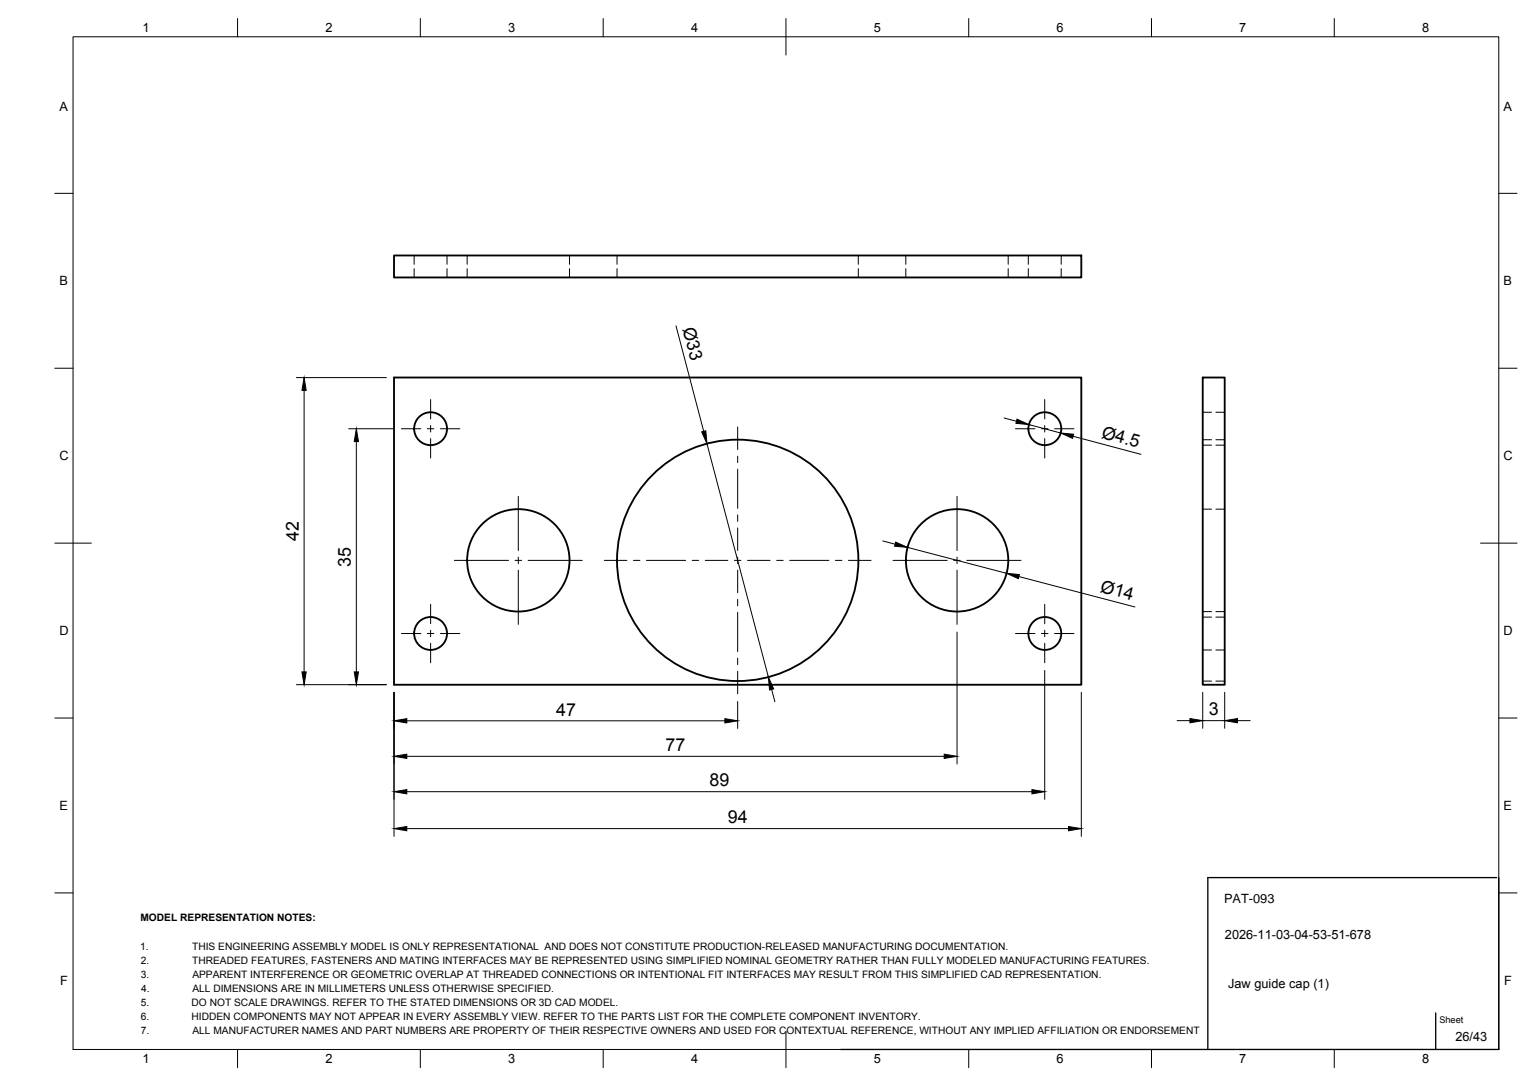
ISO-10303-21;
HEADER;
/* Generated by software containing ST-Developer
 * from STEP Tools, Inc. (www.steptools.com) 
 */

FILE_DESCRIPTION(
/* description */ ('Self-centering screw clamp'),
/* implementation_level */ '2;1');

FILE_NAME(
/* name */ 'Jaw guide cap (1).step',
/* time_stamp */ '2026-10-28T03:25:31-07:00',
/* author */ (''),
/* organization */ (''),
/* preprocessor_version */ 'ST-DEVELOPER v20.2',
/* originating_system */ 'Autodesk Translation Framework v15.17.0.0',
/* authorisation */ '');

FILE_SCHEMA (('AUTOMOTIVE_DESIGN { 1 0 10303 214 3 1 1 }'));
ENDSEC;

DATA;
#10=MECHANICAL_DESIGN_GEOMETRIC_PRESENTATION_REPRESENTATION('',(#652),#16799);
#563=SHAPE_REPRESENTATION_RELATIONSHIP('SRR','None',#17038,#604);
#604=ADVANCED_BREP_SHAPE_REPRESENTATION('',(#700),#16776);
#652=STYLED_ITEM('',(#17312),#700);
#700=MANIFOLD_SOLID_BREP('Body1',#9103);
#885=FACE_BOUND('',#2220,.T.);
#886=FACE_BOUND('',#2221,.T.);
#887=FACE_BOUND('',#2222,.T.);
#888=FACE_BOUND('',#2223,.T.);
#889=FACE_BOUND('',#2224,.T.);
#890=FACE_BOUND('',#2225,.T.);
#891=FACE_BOUND('',#2226,.T.);
#892=FACE_BOUND('',#2229,.T.);
#893=FACE_BOUND('',#2230,.T.);
#894=FACE_BOUND('',#2231,.T.);
#895=FACE_BOUND('',#2232,.T.);
#896=FACE_BOUND('',#2233,.T.);
#897=FACE_BOUND('',#2234,.T.);
#898=FACE_BOUND('',#2235,.T.);
#1140=PLANE('',#10185);
#1141=PLANE('',#10186);
#1142=PLANE('',#10187);
#1143=PLANE('',#10188);
#1144=PLANE('',#10189);
#1145=PLANE('',#10190);
#1540=FACE_OUTER_BOUND('',#2211,.T.);
#1541=FACE_OUTER_BOUND('',#2212,.T.);
#1542=FACE_OUTER_BOUND('',#2213,.T.);
#1543=FACE_OUTER_BOUND('',#2214,.T.);
#1544=FACE_OUTER_BOUND('',#2215,.T.);
#1545=FACE_OUTER_BOUND('',#2216,.T.);
#1546=FACE_OUTER_BOUND('',#2217,.T.);
#1547=FACE_OUTER_BOUND('',#2218,.T.);
#1548=FACE_OUTER_BOUND('',#2219,.T.);
#1549=FACE_OUTER_BOUND('',#2227,.T.);
#1550=FACE_OUTER_BOUND('',#2228,.T.);
#1551=FACE_OUTER_BOUND('',#2236,.T.);
#1552=FACE_OUTER_BOUND('',#2237,.T.);
#2211=EDGE_LOOP('',(#7359,#7360,#7361,#7362));
#2212=EDGE_LOOP('',(#7363,#7364,#7365,#7366));
#2213=EDGE_LOOP('',(#7367,#7368,#7369,#7370));
#2214=EDGE_LOOP('',(#7371,#7372,#7373,#7374));
#2215=EDGE_LOOP('',(#7375,#7376,#7377,#7378));
#2216=EDGE_LOOP('',(#7379,#7380,#7381,#7382));
#2217=EDGE_LOOP('',(#7383,#7384,#7385,#7386));
#2218=EDGE_LOOP('',(#7387,#7388,#7389,#7390));
#2219=EDGE_LOOP('',(#7391,#7392,#7393,#7394));
#2220=EDGE_LOOP('',(#7395));
#2221=EDGE_LOOP('',(#7396));
#2222=EDGE_LOOP('',(#7397));
#2223=EDGE_LOOP('',(#7398));
#2224=EDGE_LOOP('',(#7399));
#2225=EDGE_LOOP('',(#7400));
#2226=EDGE_LOOP('',(#7401));
#2227=EDGE_LOOP('',(#7402,#7403,#7404,#7405));
#2228=EDGE_LOOP('',(#7406,#7407,#7408,#7409));
#2229=EDGE_LOOP('',(#7410));
#2230=EDGE_LOOP('',(#7411));
#2231=EDGE_LOOP('',(#7412));
#2232=EDGE_LOOP('',(#7413));
#2233=EDGE_LOOP('',(#7414));
#2234=EDGE_LOOP('',(#7415));
#2235=EDGE_LOOP('',(#7416));
#2236=EDGE_LOOP('',(#7417,#7418,#7419,#7420));
#2237=EDGE_LOOP('',(#7421,#7422,#7423,#7424));
#2886=LINE('',#15393,#3459);
#2887=LINE('',#15399,#3460);
#2888=LINE('',#15405,#3461);
#2889=LINE('',#15411,#3462);
#2890=LINE('',#15417,#3463);
#2891=LINE('',#15423,#3464);
#2892=LINE('',#15429,#3465);
#2893=LINE('',#15434,#3466);
#2894=LINE('',#15436,#3467);
#2895=LINE('',#15438,#3468);
#2896=LINE('',#15439,#3469);
#2897=LINE('',#15442,#3470);
#2898=LINE('',#15444,#3471);
#2899=LINE('',#15445,#3472);
#2900=LINE('',#15448,#3473);
#2901=LINE('',#15450,#3474);
#2902=LINE('',#15451,#3475);
#2903=LINE('',#15453,#3476);
#2904=LINE('',#15454,#3477);
#3459=VECTOR('',#12239,0.225);
#3460=VECTOR('',#12246,0.225);
#3461=VECTOR('',#12253,0.225);
#3462=VECTOR('',#12260,0.225);
#3463=VECTOR('',#12267,1.65);
#3464=VECTOR('',#12274,0.7);
#3465=VECTOR('',#12281,0.7);
#3466=VECTOR('',#12286,1.);
#3467=VECTOR('',#12287,1.);
#3468=VECTOR('',#12288,1.);
#3469=VECTOR('',#12289,1.);
#3470=VECTOR('',#12292,1.);
#3471=VECTOR('',#12293,1.);
#3472=VECTOR('',#12294,1.);
#3473=VECTOR('',#12297,1.);
#3474=VECTOR('',#12298,1.);
#3475=VECTOR('',#12299,1.);
#3476=VECTOR('',#12302,1.);
#3477=VECTOR('',#12303,1.);
#4012=CIRCLE('',#10165,0.225);
#4013=CIRCLE('',#10166,0.225);
#4014=CIRCLE('',#10168,0.225);
#4015=CIRCLE('',#10169,0.225);
#4016=CIRCLE('',#10171,0.225);
#4017=CIRCLE('',#10172,0.225);
#4018=CIRCLE('',#10174,0.225);
#4019=CIRCLE('',#10175,0.225);
#4020=CIRCLE('',#10177,1.65);
#4021=CIRCLE('',#10178,1.65);
#4022=CIRCLE('',#10180,0.7);
#4023=CIRCLE('',#10181,0.7);
#4024=CIRCLE('',#10183,0.7);
#4025=CIRCLE('',#10184,0.7);
#4647=VERTEX_POINT('',#15390);
#4648=VERTEX_POINT('',#15392);
#4649=VERTEX_POINT('',#15396);
#4650=VERTEX_POINT('',#15398);
#4651=VERTEX_POINT('',#15402);
#4652=VERTEX_POINT('',#15404);
#4653=VERTEX_POINT('',#15408);
#4654=VERTEX_POINT('',#15410);
#4655=VERTEX_POINT('',#15414);
#4656=VERTEX_POINT('',#15416);
#4657=VERTEX_POINT('',#15420);
#4658=VERTEX_POINT('',#15422);
#4659=VERTEX_POINT('',#15426);
#4660=VERTEX_POINT('',#15428);
#4661=VERTEX_POINT('',#15432);
#4662=VERTEX_POINT('',#15433);
#4663=VERTEX_POINT('',#15435);
#4664=VERTEX_POINT('',#15437);
#4665=VERTEX_POINT('',#15441);
#4666=VERTEX_POINT('',#15443);
#4667=VERTEX_POINT('',#15447);
#4668=VERTEX_POINT('',#15449);
#5604=EDGE_CURVE('',#4647,#4647,#4012,.T.);
#5605=EDGE_CURVE('',#4647,#4648,#2886,.T.);
#5606=EDGE_CURVE('',#4648,#4648,#4013,.T.);
#5607=EDGE_CURVE('',#4649,#4649,#4014,.T.);
#5608=EDGE_CURVE('',#4649,#4650,#2887,.T.);
#5609=EDGE_CURVE('',#4650,#4650,#4015,.T.);
#5610=EDGE_CURVE('',#4651,#4651,#4016,.T.);
#5611=EDGE_CURVE('',#4651,#4652,#2888,.T.);
#5612=EDGE_CURVE('',#4652,#4652,#4017,.T.);
#5613=EDGE_CURVE('',#4653,#4653,#4018,.T.);
#5614=EDGE_CURVE('',#4653,#4654,#2889,.T.);
#5615=EDGE_CURVE('',#4654,#4654,#4019,.T.);
#5616=EDGE_CURVE('',#4655,#4655,#4020,.T.);
#5617=EDGE_CURVE('',#4655,#4656,#2890,.T.);
#5618=EDGE_CURVE('',#4656,#4656,#4021,.T.);
#5619=EDGE_CURVE('',#4657,#4657,#4022,.T.);
#5620=EDGE_CURVE('',#4657,#4658,#2891,.T.);
#5621=EDGE_CURVE('',#4658,#4658,#4023,.T.);
#5622=EDGE_CURVE('',#4659,#4659,#4024,.T.);
#5623=EDGE_CURVE('',#4659,#4660,#2892,.T.);
#5624=EDGE_CURVE('',#4660,#4660,#4025,.T.);
#5625=EDGE_CURVE('',#4661,#4662,#2893,.T.);
#5626=EDGE_CURVE('',#4662,#4663,#2894,.T.);
#5627=EDGE_CURVE('',#4664,#4663,#2895,.T.);
#5628=EDGE_CURVE('',#4661,#4664,#2896,.T.);
#5629=EDGE_CURVE('',#4665,#4661,#2897,.T.);
#5630=EDGE_CURVE('',#4666,#4664,#2898,.T.);
#5631=EDGE_CURVE('',#4665,#4666,#2899,.T.);
#5632=EDGE_CURVE('',#4667,#4665,#2900,.T.);
#5633=EDGE_CURVE('',#4668,#4666,#2901,.T.);
#5634=EDGE_CURVE('',#4667,#4668,#2902,.T.);
#5635=EDGE_CURVE('',#4662,#4667,#2903,.T.);
#5636=EDGE_CURVE('',#4663,#4668,#2904,.T.);
#7359=ORIENTED_EDGE('',*,*,#5604,.F.);
#7360=ORIENTED_EDGE('',*,*,#5605,.T.);
#7361=ORIENTED_EDGE('',*,*,#5606,.F.);
#7362=ORIENTED_EDGE('',*,*,#5605,.F.);
#7363=ORIENTED_EDGE('',*,*,#5607,.F.);
#7364=ORIENTED_EDGE('',*,*,#5608,.T.);
#7365=ORIENTED_EDGE('',*,*,#5609,.F.);
#7366=ORIENTED_EDGE('',*,*,#5608,.F.);
#7367=ORIENTED_EDGE('',*,*,#5610,.F.);
#7368=ORIENTED_EDGE('',*,*,#5611,.T.);
#7369=ORIENTED_EDGE('',*,*,#5612,.F.);
#7370=ORIENTED_EDGE('',*,*,#5611,.F.);
#7371=ORIENTED_EDGE('',*,*,#5613,.F.);
#7372=ORIENTED_EDGE('',*,*,#5614,.T.);
#7373=ORIENTED_EDGE('',*,*,#5615,.F.);
#7374=ORIENTED_EDGE('',*,*,#5614,.F.);
#7375=ORIENTED_EDGE('',*,*,#5616,.F.);
#7376=ORIENTED_EDGE('',*,*,#5617,.T.);
#7377=ORIENTED_EDGE('',*,*,#5618,.F.);
#7378=ORIENTED_EDGE('',*,*,#5617,.F.);
#7379=ORIENTED_EDGE('',*,*,#5619,.F.);
#7380=ORIENTED_EDGE('',*,*,#5620,.T.);
#7381=ORIENTED_EDGE('',*,*,#5621,.F.);
#7382=ORIENTED_EDGE('',*,*,#5620,.F.);
#7383=ORIENTED_EDGE('',*,*,#5622,.F.);
#7384=ORIENTED_EDGE('',*,*,#5623,.T.);
#7385=ORIENTED_EDGE('',*,*,#5624,.F.);
#7386=ORIENTED_EDGE('',*,*,#5623,.F.);
#7387=ORIENTED_EDGE('',*,*,#5625,.T.);
#7388=ORIENTED_EDGE('',*,*,#5626,.T.);
#7389=ORIENTED_EDGE('',*,*,#5627,.F.);
#7390=ORIENTED_EDGE('',*,*,#5628,.F.);
#7391=ORIENTED_EDGE('',*,*,#5629,.T.);
#7392=ORIENTED_EDGE('',*,*,#5628,.T.);
#7393=ORIENTED_EDGE('',*,*,#5630,.F.);
#7394=ORIENTED_EDGE('',*,*,#5631,.F.);
#7395=ORIENTED_EDGE('',*,*,#5624,.T.);
#7396=ORIENTED_EDGE('',*,*,#5621,.T.);
#7397=ORIENTED_EDGE('',*,*,#5618,.T.);
#7398=ORIENTED_EDGE('',*,*,#5615,.T.);
#7399=ORIENTED_EDGE('',*,*,#5612,.T.);
#7400=ORIENTED_EDGE('',*,*,#5609,.T.);
#7401=ORIENTED_EDGE('',*,*,#5606,.T.);
#7402=ORIENTED_EDGE('',*,*,#5632,.T.);
#7403=ORIENTED_EDGE('',*,*,#5631,.T.);
#7404=ORIENTED_EDGE('',*,*,#5633,.F.);
#7405=ORIENTED_EDGE('',*,*,#5634,.F.);
#7406=ORIENTED_EDGE('',*,*,#5635,.T.);
#7407=ORIENTED_EDGE('',*,*,#5634,.T.);
#7408=ORIENTED_EDGE('',*,*,#5636,.F.);
#7409=ORIENTED_EDGE('',*,*,#5626,.F.);
#7410=ORIENTED_EDGE('',*,*,#5622,.T.);
#7411=ORIENTED_EDGE('',*,*,#5619,.T.);
#7412=ORIENTED_EDGE('',*,*,#5616,.T.);
#7413=ORIENTED_EDGE('',*,*,#5613,.T.);
#7414=ORIENTED_EDGE('',*,*,#5610,.T.);
#7415=ORIENTED_EDGE('',*,*,#5607,.T.);
#7416=ORIENTED_EDGE('',*,*,#5604,.T.);
#7417=ORIENTED_EDGE('',*,*,#5636,.T.);
#7418=ORIENTED_EDGE('',*,*,#5633,.T.);
#7419=ORIENTED_EDGE('',*,*,#5630,.T.);
#7420=ORIENTED_EDGE('',*,*,#5627,.T.);
#7421=ORIENTED_EDGE('',*,*,#5635,.F.);
#7422=ORIENTED_EDGE('',*,*,#5625,.F.);
#7423=ORIENTED_EDGE('',*,*,#5629,.F.);
#7424=ORIENTED_EDGE('',*,*,#5632,.F.);
#8476=CYLINDRICAL_SURFACE('',#10164,0.225);
#8477=CYLINDRICAL_SURFACE('',#10167,0.225);
#8478=CYLINDRICAL_SURFACE('',#10170,0.225);
#8479=CYLINDRICAL_SURFACE('',#10173,0.225);
#8480=CYLINDRICAL_SURFACE('',#10176,1.65);
#8481=CYLINDRICAL_SURFACE('',#10179,0.7);
#8482=CYLINDRICAL_SURFACE('',#10182,0.7);
#8838=ADVANCED_FACE('',(#1540),#8476,.F.);
#8839=ADVANCED_FACE('',(#1541),#8477,.F.);
#8840=ADVANCED_FACE('',(#1542),#8478,.F.);
#8841=ADVANCED_FACE('',(#1543),#8479,.F.);
#8842=ADVANCED_FACE('',(#1544),#8480,.F.);
#8843=ADVANCED_FACE('',(#1545),#8481,.F.);
#8844=ADVANCED_FACE('',(#1546),#8482,.F.);
#8845=ADVANCED_FACE('',(#1547),#1140,.T.);
#8846=ADVANCED_FACE('',(#1548,#885,#886,#887,#888,#889,#890,#891),#1141,
 .T.);
#8847=ADVANCED_FACE('',(#1549),#1142,.T.);
#8848=ADVANCED_FACE('',(#1550,#892,#893,#894,#895,#896,#897,#898),#1143,
 .T.);
#8849=ADVANCED_FACE('',(#1551),#1144,.T.);
#8850=ADVANCED_FACE('',(#1552),#1145,.F.);
#9103=CLOSED_SHELL('',(#8838,#8839,#8840,#8841,#8842,#8843,#8844,#8845,
#8846,#8847,#8848,#8849,#8850));
#10163=AXIS2_PLACEMENT_3D('',#15388,#12233,#12234);
#10164=AXIS2_PLACEMENT_3D('',#15389,#12235,#12236);
#10165=AXIS2_PLACEMENT_3D('',#15391,#12237,#12238);
#10166=AXIS2_PLACEMENT_3D('',#15394,#12240,#12241);
#10167=AXIS2_PLACEMENT_3D('',#15395,#12242,#12243);
#10168=AXIS2_PLACEMENT_3D('',#15397,#12244,#12245);
#10169=AXIS2_PLACEMENT_3D('',#15400,#12247,#12248);
#10170=AXIS2_PLACEMENT_3D('',#15401,#12249,#12250);
#10171=AXIS2_PLACEMENT_3D('',#15403,#12251,#12252);
#10172=AXIS2_PLACEMENT_3D('',#15406,#12254,#12255);
#10173=AXIS2_PLACEMENT_3D('',#15407,#12256,#12257);
#10174=AXIS2_PLACEMENT_3D('',#15409,#12258,#12259);
#10175=AXIS2_PLACEMENT_3D('',#15412,#12261,#12262);
#10176=AXIS2_PLACEMENT_3D('',#15413,#12263,#12264);
#10177=AXIS2_PLACEMENT_3D('',#15415,#12265,#12266);
#10178=AXIS2_PLACEMENT_3D('',#15418,#12268,#12269);
#10179=AXIS2_PLACEMENT_3D('',#15419,#12270,#12271);
#10180=AXIS2_PLACEMENT_3D('',#15421,#12272,#12273);
#10181=AXIS2_PLACEMENT_3D('',#15424,#12275,#12276);
#10182=AXIS2_PLACEMENT_3D('',#15425,#12277,#12278);
#10183=AXIS2_PLACEMENT_3D('',#15427,#12279,#12280);
#10184=AXIS2_PLACEMENT_3D('',#15430,#12282,#12283);
#10185=AXIS2_PLACEMENT_3D('',#15431,#12284,#12285);
#10186=AXIS2_PLACEMENT_3D('',#15440,#12290,#12291);
#10187=AXIS2_PLACEMENT_3D('',#15446,#12295,#12296);
#10188=AXIS2_PLACEMENT_3D('',#15452,#12300,#12301);
#10189=AXIS2_PLACEMENT_3D('',#15455,#12304,#12305);
#10190=AXIS2_PLACEMENT_3D('',#15456,#12306,#12307);
#12233=DIRECTION('axis',(0.,0.,1.));
#12234=DIRECTION('refdir',(1.,0.,0.));
#12235=DIRECTION('center_axis',(1.,0.,0.));
#12236=DIRECTION('ref_axis',(0.,0.,-1.));
#12237=DIRECTION('center_axis',(1.,0.,0.));
#12238=DIRECTION('ref_axis',(0.,0.,-1.));
#12239=DIRECTION('',(1.,0.,0.));
#12240=DIRECTION('center_axis',(-1.,0.,0.));
#12241=DIRECTION('ref_axis',(0.,0.,-1.));
#12242=DIRECTION('center_axis',(1.,0.,0.));
#12243=DIRECTION('ref_axis',(0.,0.,-1.));
#12244=DIRECTION('center_axis',(1.,0.,0.));
#12245=DIRECTION('ref_axis',(0.,0.,-1.));
#12246=DIRECTION('',(1.,0.,0.));
#12247=DIRECTION('center_axis',(-1.,0.,0.));
#12248=DIRECTION('ref_axis',(0.,0.,-1.));
#12249=DIRECTION('center_axis',(1.,0.,0.));
#12250=DIRECTION('ref_axis',(0.,0.,-1.));
#12251=DIRECTION('center_axis',(1.,0.,0.));
#12252=DIRECTION('ref_axis',(0.,0.,-1.));
#12253=DIRECTION('',(1.,0.,0.));
#12254=DIRECTION('center_axis',(-1.,0.,0.));
#12255=DIRECTION('ref_axis',(0.,0.,-1.));
#12256=DIRECTION('center_axis',(1.,0.,0.));
#12257=DIRECTION('ref_axis',(0.,0.,-1.));
#12258=DIRECTION('center_axis',(1.,0.,0.));
#12259=DIRECTION('ref_axis',(0.,0.,-1.));
#12260=DIRECTION('',(1.,0.,0.));
#12261=DIRECTION('center_axis',(-1.,0.,0.));
#12262=DIRECTION('ref_axis',(0.,0.,-1.));
#12263=DIRECTION('center_axis',(1.,0.,0.));
#12264=DIRECTION('ref_axis',(0.,0.,-1.));
#12265=DIRECTION('center_axis',(1.,0.,0.));
#12266=DIRECTION('ref_axis',(0.,0.,-1.));
#12267=DIRECTION('',(1.,0.,0.));
#12268=DIRECTION('center_axis',(-1.,0.,0.));
#12269=DIRECTION('ref_axis',(0.,0.,-1.));
#12270=DIRECTION('center_axis',(1.,0.,0.));
#12271=DIRECTION('ref_axis',(0.,0.,-1.));
#12272=DIRECTION('center_axis',(1.,0.,0.));
#12273=DIRECTION('ref_axis',(0.,0.,-1.));
#12274=DIRECTION('',(1.,0.,0.));
#12275=DIRECTION('center_axis',(-1.,0.,0.));
#12276=DIRECTION('ref_axis',(0.,0.,-1.));
#12277=DIRECTION('center_axis',(1.,0.,0.));
#12278=DIRECTION('ref_axis',(0.,0.,-1.));
#12279=DIRECTION('center_axis',(1.,0.,0.));
#12280=DIRECTION('ref_axis',(0.,0.,-1.));
#12281=DIRECTION('',(1.,0.,0.));
#12282=DIRECTION('center_axis',(-1.,0.,0.));
#12283=DIRECTION('ref_axis',(0.,0.,-1.));
#12284=DIRECTION('center_axis',(0.,1.,0.));
#12285=DIRECTION('ref_axis',(-1.,0.,0.));
#12286=DIRECTION('',(-1.,0.,0.));
#12287=DIRECTION('',(0.,0.,1.));
#12288=DIRECTION('',(-1.,0.,0.));
#12289=DIRECTION('',(0.,0.,1.));
#12290=DIRECTION('center_axis',(1.,0.,0.));
#12291=DIRECTION('ref_axis',(0.,1.,0.));
#12292=DIRECTION('',(0.,1.,0.));
#12293=DIRECTION('',(0.,1.,0.));
#12294=DIRECTION('',(0.,0.,1.));
#12295=DIRECTION('center_axis',(0.,-1.,0.));
#12296=DIRECTION('ref_axis',(1.,0.,0.));
#12297=DIRECTION('',(1.,0.,0.));
#12298=DIRECTION('',(1.,0.,0.));
#12299=DIRECTION('',(0.,0.,1.));
#12300=DIRECTION('center_axis',(-1.,0.,0.));
#12301=DIRECTION('ref_axis',(0.,-1.,0.));
#12302=DIRECTION('',(0.,-1.,0.));
#12303=DIRECTION('',(0.,-1.,0.));
#12304=DIRECTION('center_axis',(0.,0.,1.));
#12305=DIRECTION('ref_axis',(1.,0.,0.));
#12306=DIRECTION('center_axis',(0.,0.,1.));
#12307=DIRECTION('ref_axis',(1.,0.,0.));
#15388=CARTESIAN_POINT('',(0.,0.,0.));
#15389=CARTESIAN_POINT('Origin',(-5.6,4.2,3.));
#15390=CARTESIAN_POINT('',(-5.5,4.2,3.225));
#15391=CARTESIAN_POINT('Origin',(-5.5,4.2,3.));
#15392=CARTESIAN_POINT('',(-5.2,4.2,3.225));
#15393=CARTESIAN_POINT('',(-5.6,4.2,3.225));
#15394=CARTESIAN_POINT('Origin',(-5.2,4.2,3.));
#15395=CARTESIAN_POINT('Origin',(-5.6,-4.2,5.8));
#15396=CARTESIAN_POINT('',(-5.5,-4.2,6.025));
#15397=CARTESIAN_POINT('Origin',(-5.5,-4.2,5.8));
#15398=CARTESIAN_POINT('',(-5.2,-4.2,6.025));
#15399=CARTESIAN_POINT('',(-5.6,-4.2,6.025));
#15400=CARTESIAN_POINT('Origin',(-5.2,-4.2,5.8));
#15401=CARTESIAN_POINT('Origin',(-5.6,-4.2,3.));
#15402=CARTESIAN_POINT('',(-5.5,-4.2,3.225));
#15403=CARTESIAN_POINT('Origin',(-5.5,-4.2,3.));
#15404=CARTESIAN_POINT('',(-5.2,-4.2,3.225));
#15405=CARTESIAN_POINT('',(-5.6,-4.2,3.225));
#15406=CARTESIAN_POINT('Origin',(-5.2,-4.2,3.));
#15407=CARTESIAN_POINT('Origin',(-5.6,4.2,5.8));
#15408=CARTESIAN_POINT('',(-5.5,4.2,6.025));
#15409=CARTESIAN_POINT('Origin',(-5.5,4.2,5.8));
#15410=CARTESIAN_POINT('',(-5.2,4.2,6.025));
#15411=CARTESIAN_POINT('',(-5.6,4.2,6.025));
#15412=CARTESIAN_POINT('Origin',(-5.2,4.2,5.8));
#15413=CARTESIAN_POINT('Origin',(-5.6,0.,4.));
#15414=CARTESIAN_POINT('',(-5.5,-2.02066721859313E-16,5.65));
#15415=CARTESIAN_POINT('Origin',(-5.5,0.,4.));
#15416=CARTESIAN_POINT('',(-5.2,2.02066721859313E-16,5.65));
#15417=CARTESIAN_POINT('',(-5.6,-2.02066721859313E-16,5.65));
#15418=CARTESIAN_POINT('Origin',(-5.2,0.,4.));
#15419=CARTESIAN_POINT('Origin',(-5.6,-3.,4.));
#15420=CARTESIAN_POINT('',(-5.5,-3.,4.7));
#15421=CARTESIAN_POINT('Origin',(-5.5,-3.,4.));
#15422=CARTESIAN_POINT('',(-5.2,-3.,4.7));
#15423=CARTESIAN_POINT('',(-5.6,-3.,4.7));
#15424=CARTESIAN_POINT('Origin',(-5.2,-3.,4.));
#15425=CARTESIAN_POINT('Origin',(-5.6,3.,4.));
#15426=CARTESIAN_POINT('',(-5.5,3.,4.7));
#15427=CARTESIAN_POINT('Origin',(-5.5,3.,4.));
#15428=CARTESIAN_POINT('',(-5.2,3.,4.7));
#15429=CARTESIAN_POINT('',(-5.6,3.,4.7));
#15430=CARTESIAN_POINT('Origin',(-5.2,3.,4.));
#15431=CARTESIAN_POINT('Origin',(-5.2,4.7,2.3));
#15432=CARTESIAN_POINT('',(-5.2,4.7,2.3));
#15433=CARTESIAN_POINT('',(-5.5,4.7,2.3));
#15434=CARTESIAN_POINT('',(-5.2,4.7,2.3));
#15435=CARTESIAN_POINT('',(-5.5,4.7,6.5));
#15436=CARTESIAN_POINT('',(-5.5,4.7,2.3));
#15437=CARTESIAN_POINT('',(-5.2,4.7,6.5));
#15438=CARTESIAN_POINT('',(-5.2,4.7,6.5));
#15439=CARTESIAN_POINT('',(-5.2,4.7,2.3));
#15440=CARTESIAN_POINT('Origin',(-5.2,-4.7,2.3));
#15441=CARTESIAN_POINT('',(-5.2,-4.7,2.3));
#15442=CARTESIAN_POINT('',(-5.2,-4.7,2.3));
#15443=CARTESIAN_POINT('',(-5.2,-4.7,6.5));
#15444=CARTESIAN_POINT('',(-5.2,-4.7,6.5));
#15445=CARTESIAN_POINT('',(-5.2,-4.7,2.3));
#15446=CARTESIAN_POINT('Origin',(-5.5,-4.7,2.3));
#15447=CARTESIAN_POINT('',(-5.5,-4.7,2.3));
#15448=CARTESIAN_POINT('',(-5.5,-4.7,2.3));
#15449=CARTESIAN_POINT('',(-5.5,-4.7,6.5));
#15450=CARTESIAN_POINT('',(-5.5,-4.7,6.5));
#15451=CARTESIAN_POINT('',(-5.5,-4.7,2.3));
#15452=CARTESIAN_POINT('Origin',(-5.5,4.7,2.3));
#15453=CARTESIAN_POINT('',(-5.5,4.7,2.3));
#15454=CARTESIAN_POINT('',(-5.5,4.7,6.5));
#15455=CARTESIAN_POINT('Origin',(-5.35,0.,6.5));
#15456=CARTESIAN_POINT('Origin',(-5.35,0.,2.3));
#16727=UNCERTAINTY_MEASURE_WITH_UNIT(LENGTH_MEASURE(0.001),#16800,
'DISTANCE_ACCURACY_VALUE',
'Maximum model space distance between geometric entities at asserted c
onnectivities');
#16750=UNCERTAINTY_MEASURE_WITH_UNIT(LENGTH_MEASURE(0.001),#16800,
'DISTANCE_ACCURACY_VALUE',
'Maximum model space distance between geometric entities at asserted c
onnectivities');
#16776=(
GEOMETRIC_REPRESENTATION_CONTEXT(3)
GLOBAL_UNCERTAINTY_ASSIGNED_CONTEXT((#16727))
GLOBAL_UNIT_ASSIGNED_CONTEXT((#16800,#16802,#16803))
REPRESENTATION_CONTEXT('','3D')
);
#16799=(
GEOMETRIC_REPRESENTATION_CONTEXT(3)
GLOBAL_UNCERTAINTY_ASSIGNED_CONTEXT((#16750))
GLOBAL_UNIT_ASSIGNED_CONTEXT((#16800,#16802,#16803))
REPRESENTATION_CONTEXT('','3D')
);
#16800=(
LENGTH_UNIT()
NAMED_UNIT(*)
SI_UNIT(.CENTI.,.METRE.)
);
#16802=(
NAMED_UNIT(*)
PLANE_ANGLE_UNIT()
SI_UNIT($,.RADIAN.)
);
#16803=(
NAMED_UNIT(*)
SI_UNIT($,.STERADIAN.)
SOLID_ANGLE_UNIT()
);
#16829=SHAPE_DEFINITION_REPRESENTATION(#16882,#17038);
#16882=PRODUCT_DEFINITION_SHAPE('',$,#17087);
#17038=SHAPE_REPRESENTATION('',(#10163),#16776);
#17061=PRODUCT_DEFINITION_CONTEXT('part definition',#17207,'design');
#17087=PRODUCT_DEFINITION('Jaw guide cap (1)','Jaw guide cap (1)',#17135,
#17061);
#17135=PRODUCT_DEFINITION_FORMATION('',$,#17234);
#17207=APPLICATION_CONTEXT(
'Core Data for Automotive Mechanical Design Process');
#17208=PRODUCT_CONTEXT('part definition',#17207,'mechanical');
#17234=PRODUCT('Jaw guide cap (1)','Jaw guide cap (1)','Jaw guide cap (1)',(#17208));
#17306=COLOUR_RGB('Light Blue',0.38,0.62,0.78);
#17307=FILL_AREA_STYLE_COLOUR('',#17306);
#17308=FILL_AREA_STYLE('',(#17307));
#17309=SURFACE_STYLE_FILL_AREA(#17308);
#17310=SURFACE_SIDE_STYLE('',(#17309));
#17311=SURFACE_STYLE_USAGE(.BOTH.,#17310);
#17312=PRESENTATION_STYLE_ASSIGNMENT((#17311));
ENDSEC;
END-ISO-10303-21;
